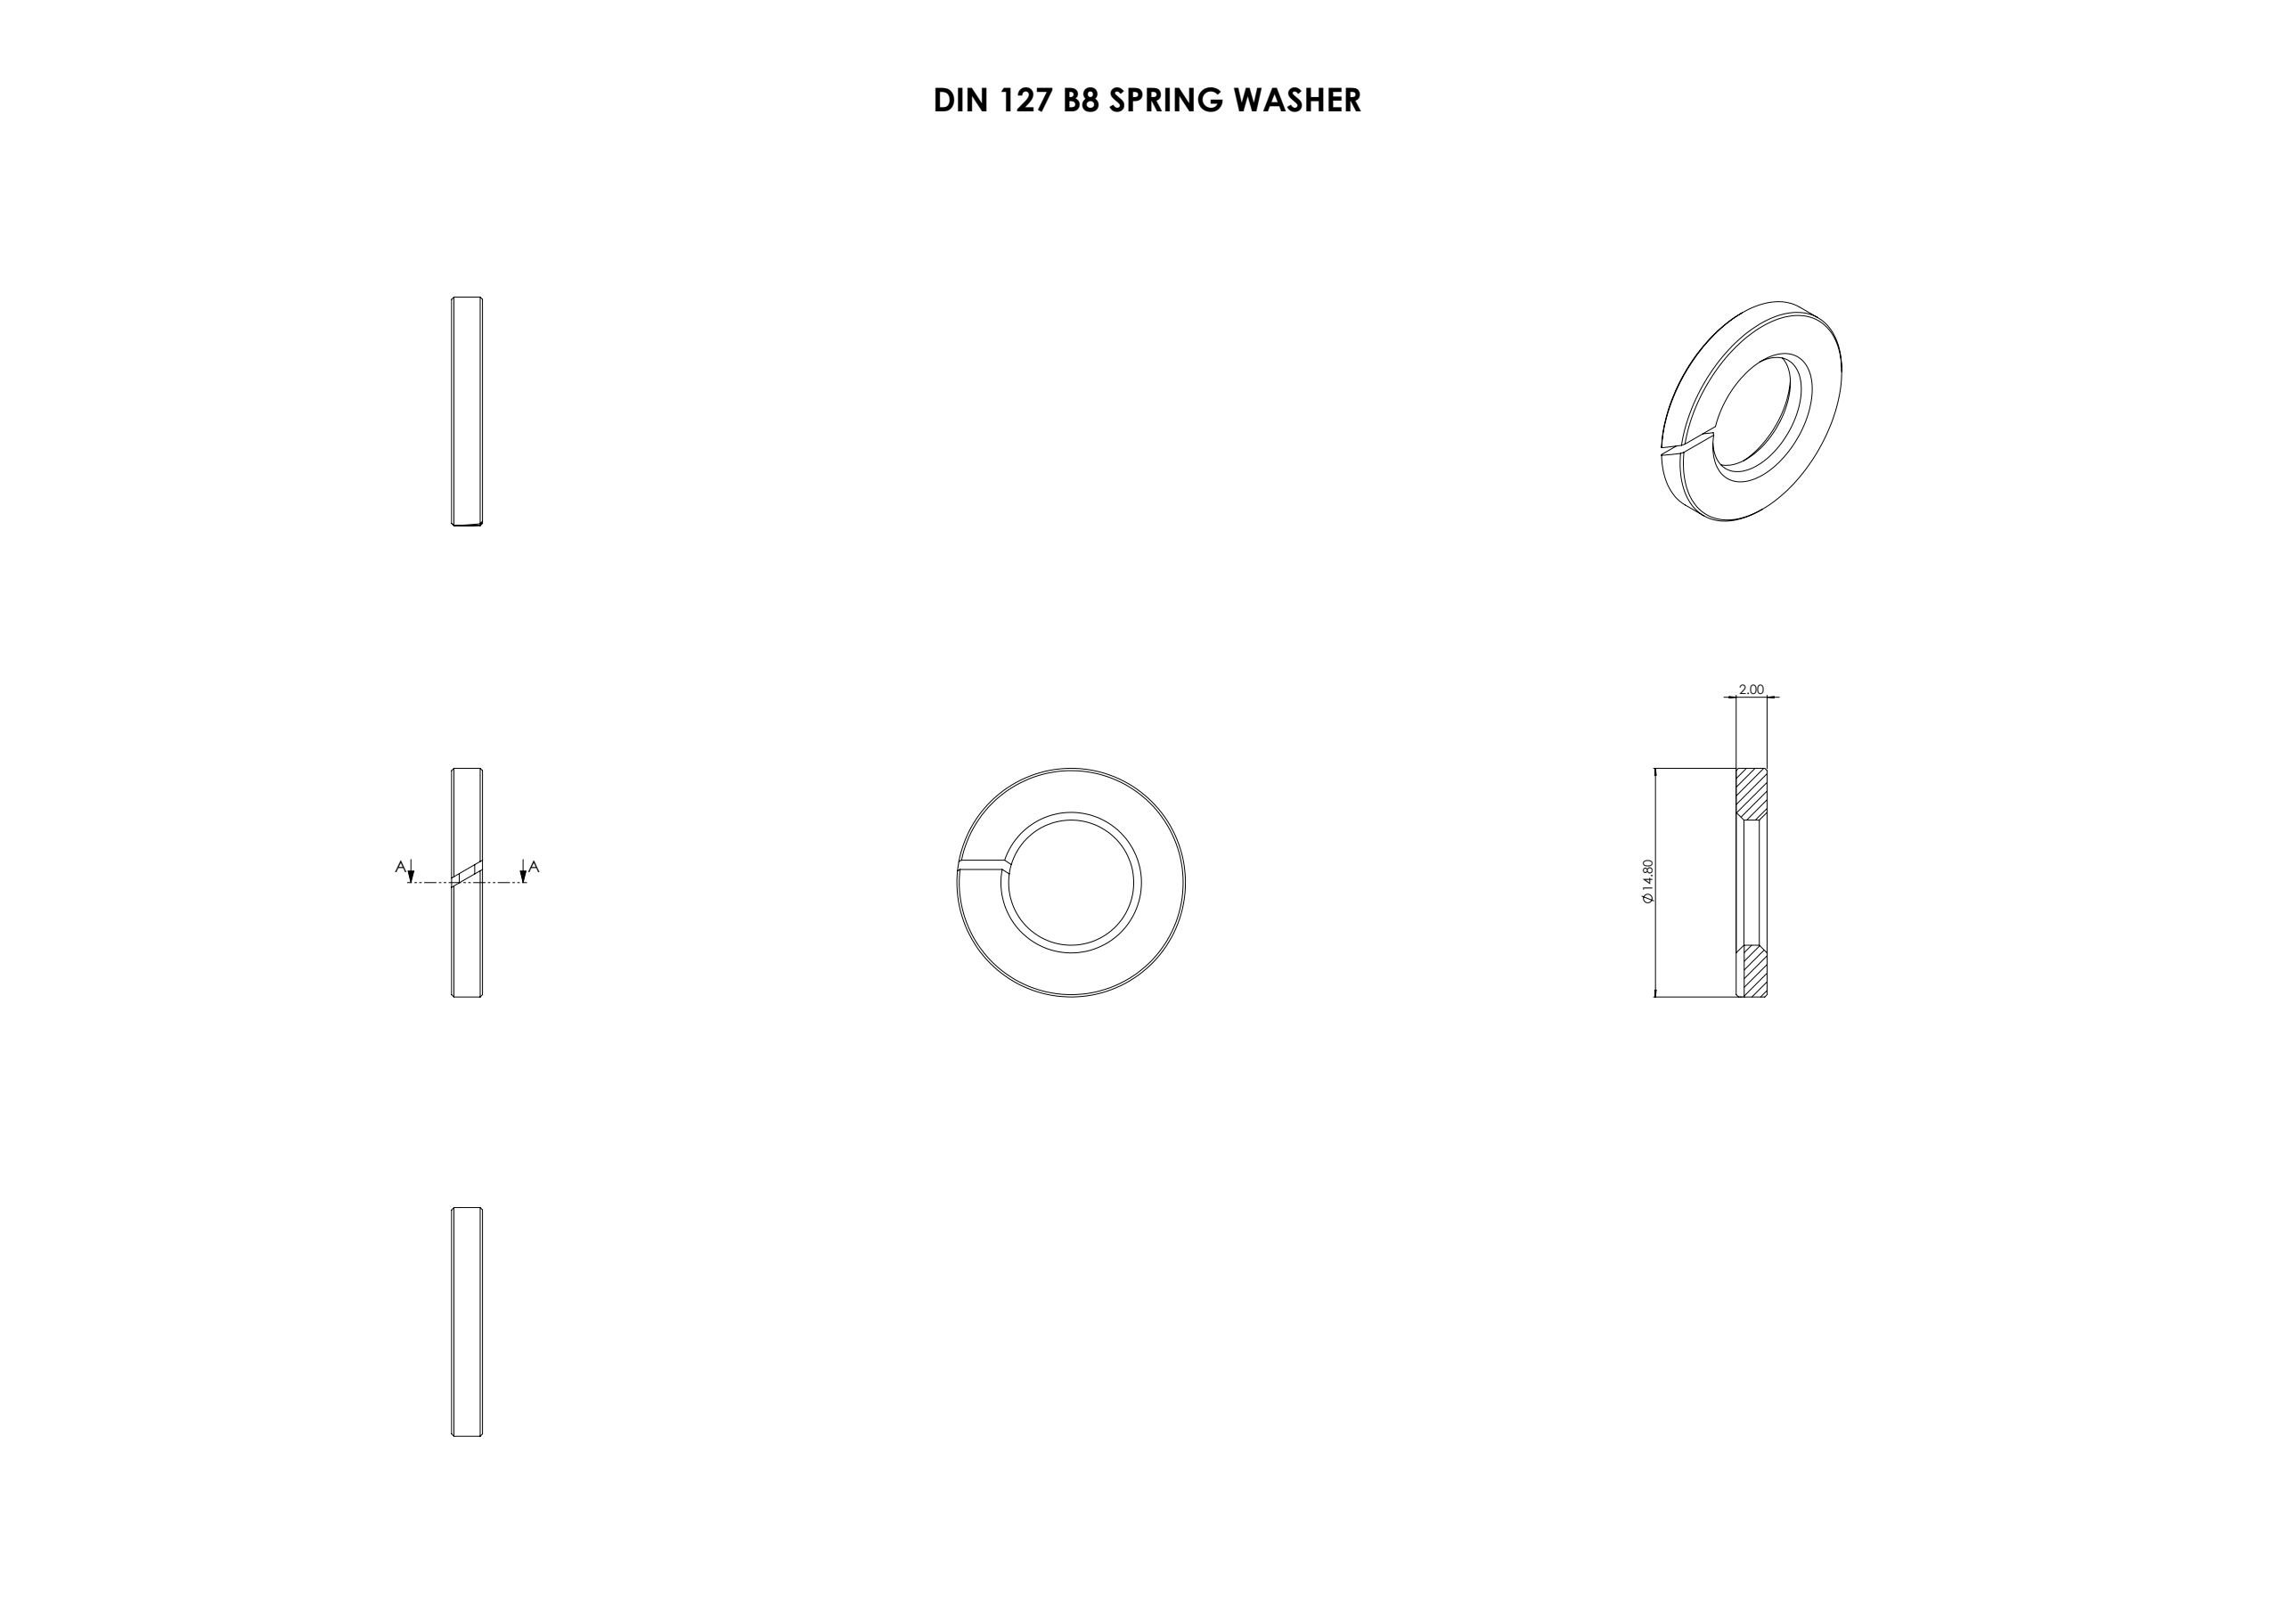
ISO-10303-21;
HEADER;
/* Generated by software containing ST-Developer
 * from STEP Tools, Inc. (www.steptools.com) 
 */

FILE_DESCRIPTION(
/* description */ (''),
/* implementation_level */ '2;1');

FILE_NAME(
/* name */ '13_DIN_127_B8_Spring_Washer.step',
/* time_stamp */ '2026-10-11T08:27:52-07:00',
/* author */ (''),
/* organization */ (''),
/* preprocessor_version */ 'ST-DEVELOPER v20.2',
/* originating_system */ 'Autodesk Translation Framework v15.15.0.0',
/* authorisation */ '');

FILE_SCHEMA (('AUTOMOTIVE_DESIGN { 1 0 10303 214 3 1 1 }'));
ENDSEC;

DATA;
#10=MECHANICAL_DESIGN_GEOMETRIC_PRESENTATION_REPRESENTATION('',(#931),#94301);
#903=SHAPE_REPRESENTATION_RELATIONSHIP('SRR','None',#94383,#917);
#917=ADVANCED_BREP_SHAPE_REPRESENTATION('',(#945),#94299);
#931=STYLED_ITEM('',(#94588),#945);
#945=MANIFOLD_SOLID_BREP('Body1',#51030);
#1284=CYLINDRICAL_SURFACE('',#55289,7.4);
#1285=CYLINDRICAL_SURFACE('',#55301,7.4);
#1286=CYLINDRICAL_SURFACE('',#55309,4.05);
#2156=ELLIPSE('',#55291,14.8,7.4);
#2157=ELLIPSE('',#55294,14.8,7.4);
#2158=ELLIPSE('',#55295,8.1,4.05);
#2159=ELLIPSE('',#55297,8.1,4.05);
#6672=LINE('',#94082,#11200);
#6673=LINE('',#94095,#11201);
#6674=LINE('',#94107,#11202);
#6675=LINE('',#94126,#11203);
#6676=LINE('',#94134,#11204);
#11200=VECTOR('',#68086,7.4);
#11201=VECTOR('',#68095,10.);
#11202=VECTOR('',#68098,10.);
#11203=VECTOR('',#68105,10.);
#11204=VECTOR('',#68106,10.);
#13237=PLANE('',#55293);
#13238=PLANE('',#55296);
#13239=PLANE('',#55305);
#13240=PLANE('',#55313);
#15907=FACE_OUTER_BOUND('',#18672,.T.);
#15908=FACE_OUTER_BOUND('',#18673,.T.);
#15909=FACE_OUTER_BOUND('',#18674,.T.);
#15910=FACE_OUTER_BOUND('',#18675,.T.);
#15911=FACE_OUTER_BOUND('',#18676,.T.);
#15912=FACE_OUTER_BOUND('',#18677,.T.);
#15913=FACE_OUTER_BOUND('',#18678,.T.);
#15914=FACE_OUTER_BOUND('',#18679,.T.);
#15915=FACE_OUTER_BOUND('',#18680,.T.);
#15916=FACE_OUTER_BOUND('',#18681,.T.);
#15917=FACE_OUTER_BOUND('',#18682,.T.);
#18672=EDGE_LOOP('',(#48003,#48004,#48005,#48006));
#18673=EDGE_LOOP('',(#48007,#48008,#48009,#48010,#48011,#48012,#48013,#48014));
#18674=EDGE_LOOP('',(#48015,#48016,#48017,#48018,#48019,#48020,#48021,#48022));
#18675=EDGE_LOOP('',(#48023,#48024,#48025,#48026,#48027));
#18676=EDGE_LOOP('',(#48028,#48029,#48030,#48031));
#18677=EDGE_LOOP('',(#48032,#48033,#48034,#48035,#48036));
#18678=EDGE_LOOP('',(#48037,#48038,#48039,#48040));
#18679=EDGE_LOOP('',(#48041,#48042,#48043,#48044));
#18680=EDGE_LOOP('',(#48045,#48046,#48047,#48048));
#18681=EDGE_LOOP('',(#48049,#48050,#48051,#48052));
#18682=EDGE_LOOP('',(#48053,#48054,#48055,#48056));
#19554=(
BOUNDED_CURVE()
B_SPLINE_CURVE(2,(#94091,#94092,#94093),.UNSPECIFIED.,.F.,.F.)
B_SPLINE_CURVE_WITH_KNOTS((3,3),(0.,0.0721484594100608),.UNSPECIFIED.)
CURVE()
GEOMETRIC_REPRESENTATION_ITEM()
RATIONAL_B_SPLINE_CURVE((1.,1.00124478006548,1.))
REPRESENTATION_ITEM('')
);
#19555=(
BOUNDED_CURVE()
B_SPLINE_CURVE(2,(#94097,#94098,#94099),.UNSPECIFIED.,.F.,.F.)
B_SPLINE_CURVE_WITH_KNOTS((3,3),(0.,0.0242606382665389),.UNSPECIFIED.)
CURVE()
GEOMETRIC_REPRESENTATION_ITEM()
RATIONAL_B_SPLINE_CURVE((1.,1.00003629689575,1.))
REPRESENTATION_ITEM('')
);
#19556=(
BOUNDED_CURVE()
B_SPLINE_CURVE(2,(#94103,#94104,#94105),.UNSPECIFIED.,.F.,.F.)
B_SPLINE_CURVE_WITH_KNOTS((3,3),(0.,0.022659739228849),.UNSPECIFIED.)
CURVE()
GEOMETRIC_REPRESENTATION_ITEM()
RATIONAL_B_SPLINE_CURVE((1.,1.00003502487514,1.))
REPRESENTATION_ITEM('')
);
#19557=(
BOUNDED_CURVE()
B_SPLINE_CURVE(2,(#94109,#94110,#94111),.UNSPECIFIED.,.F.,.F.)
B_SPLINE_CURVE_WITH_KNOTS((3,3),(0.,0.0785853165973684),.UNSPECIFIED.)
CURVE()
GEOMETRIC_REPRESENTATION_ITEM()
RATIONAL_B_SPLINE_CURVE((1.,1.00114268434673,1.))
REPRESENTATION_ITEM('')
);
#19558=(
BOUNDED_CURVE()
B_SPLINE_CURVE(2,(#94116,#94117,#94118),.UNSPECIFIED.,.F.,.F.)
B_SPLINE_CURVE_WITH_KNOTS((3,3),(0.,0.0737421516508094),.UNSPECIFIED.)
CURVE()
GEOMETRIC_REPRESENTATION_ITEM()
RATIONAL_B_SPLINE_CURVE((1.,1.00116107240881,1.))
REPRESENTATION_ITEM('')
);
#19559=(
BOUNDED_CURVE()
B_SPLINE_CURVE(2,(#94122,#94123,#94124),.UNSPECIFIED.,.F.,.F.)
B_SPLINE_CURVE_WITH_KNOTS((3,3),(0.,0.0757335241689913),.UNSPECIFIED.)
CURVE()
GEOMETRIC_REPRESENTATION_ITEM()
RATIONAL_B_SPLINE_CURVE((1.,1.00113125487949,1.))
REPRESENTATION_ITEM('')
);
#19560=(
BOUNDED_CURVE()
B_SPLINE_CURVE(2,(#94127,#94128,#94129),.UNSPECIFIED.,.F.,.F.)
B_SPLINE_CURVE_WITH_KNOTS((3,3),(0.,0.0231191378819049),.UNSPECIFIED.)
CURVE()
GEOMETRIC_REPRESENTATION_ITEM()
RATIONAL_B_SPLINE_CURVE((1.,1.00003499126588,1.))
REPRESENTATION_ITEM('')
);
#19561=(
BOUNDED_CURVE()
B_SPLINE_CURVE(2,(#94131,#94132,#94133),.UNSPECIFIED.,.F.,.F.)
B_SPLINE_CURVE_WITH_KNOTS((3,3),(0.,0.0236194283361202),.UNSPECIFIED.)
CURVE()
GEOMETRIC_REPRESENTATION_ITEM()
RATIONAL_B_SPLINE_CURVE((1.,1.0000353828725,1.))
REPRESENTATION_ITEM('')
);
#20308=CIRCLE('',#55290,7.4);
#20309=CIRCLE('',#55292,7.4);
#20310=CIRCLE('',#55299,7.4);
#20311=CIRCLE('',#55300,7.25);
#20312=CIRCLE('',#55302,7.4);
#20313=CIRCLE('',#55304,7.25);
#20314=CIRCLE('',#55306,4.55);
#20315=CIRCLE('',#55308,4.05);
#20316=CIRCLE('',#55310,4.05);
#20317=CIRCLE('',#55312,4.55);
#25285=VERTEX_POINT('',#94080);
#25286=VERTEX_POINT('',#94081);
#25287=VERTEX_POINT('',#94083);
#25288=VERTEX_POINT('',#94085);
#25289=VERTEX_POINT('',#94089);
#25290=VERTEX_POINT('',#94090);
#25291=VERTEX_POINT('',#94094);
#25292=VERTEX_POINT('',#94096);
#25293=VERTEX_POINT('',#94100);
#25294=VERTEX_POINT('',#94102);
#25295=VERTEX_POINT('',#94106);
#25296=VERTEX_POINT('',#94108);
#25297=VERTEX_POINT('',#94114);
#25298=VERTEX_POINT('',#94115);
#25299=VERTEX_POINT('',#94119);
#25300=VERTEX_POINT('',#94121);
#25301=VERTEX_POINT('',#94125);
#25302=VERTEX_POINT('',#94130);
#32863=EDGE_CURVE('',#25285,#25286,#6672,.T.);
#32864=EDGE_CURVE('',#25287,#25285,#20308,.T.);
#32865=EDGE_CURVE('',#25287,#25288,#2156,.T.);
#32866=EDGE_CURVE('',#25286,#25288,#20309,.T.);
#32867=EDGE_CURVE('',#25289,#25290,#19554,.T.);
#32868=EDGE_CURVE('',#25291,#25289,#6673,.T.);
#32869=EDGE_CURVE('',#25292,#25291,#19555,.T.);
#32870=EDGE_CURVE('',#25293,#25292,#2157,.T.);
#32871=EDGE_CURVE('',#25294,#25293,#19556,.T.);
#32872=EDGE_CURVE('',#25295,#25294,#6674,.T.);
#32873=EDGE_CURVE('',#25296,#25295,#19557,.T.);
#32874=EDGE_CURVE('',#25290,#25296,#2158,.T.);
#32875=EDGE_CURVE('',#25297,#25298,#19558,.T.);
#32876=EDGE_CURVE('',#25299,#25297,#2159,.T.);
#32877=EDGE_CURVE('',#25300,#25299,#19559,.T.);
#32878=EDGE_CURVE('',#25301,#25300,#6675,.T.);
#32879=EDGE_CURVE('',#25288,#25301,#19560,.T.);
#32880=EDGE_CURVE('',#25302,#25287,#19561,.T.);
#32881=EDGE_CURVE('',#25298,#25302,#6676,.T.);
#32882=EDGE_CURVE('',#25293,#25286,#20310,.T.);
#32883=EDGE_CURVE('',#25301,#25294,#20311,.T.);
#32884=EDGE_CURVE('',#25285,#25292,#20312,.T.);
#32885=EDGE_CURVE('',#25291,#25302,#20313,.T.);
#32886=EDGE_CURVE('',#25298,#25289,#20314,.T.);
#32887=EDGE_CURVE('',#25290,#25297,#20315,.T.);
#32888=EDGE_CURVE('',#25299,#25296,#20316,.T.);
#32889=EDGE_CURVE('',#25295,#25300,#20317,.T.);
#48003=ORIENTED_EDGE('',*,*,#32863,.F.);
#48004=ORIENTED_EDGE('',*,*,#32864,.F.);
#48005=ORIENTED_EDGE('',*,*,#32865,.T.);
#48006=ORIENTED_EDGE('',*,*,#32866,.F.);
#48007=ORIENTED_EDGE('',*,*,#32867,.F.);
#48008=ORIENTED_EDGE('',*,*,#32868,.F.);
#48009=ORIENTED_EDGE('',*,*,#32869,.F.);
#48010=ORIENTED_EDGE('',*,*,#32870,.F.);
#48011=ORIENTED_EDGE('',*,*,#32871,.F.);
#48012=ORIENTED_EDGE('',*,*,#32872,.F.);
#48013=ORIENTED_EDGE('',*,*,#32873,.F.);
#48014=ORIENTED_EDGE('',*,*,#32874,.F.);
#48015=ORIENTED_EDGE('',*,*,#32875,.F.);
#48016=ORIENTED_EDGE('',*,*,#32876,.F.);
#48017=ORIENTED_EDGE('',*,*,#32877,.F.);
#48018=ORIENTED_EDGE('',*,*,#32878,.F.);
#48019=ORIENTED_EDGE('',*,*,#32879,.F.);
#48020=ORIENTED_EDGE('',*,*,#32865,.F.);
#48021=ORIENTED_EDGE('',*,*,#32880,.F.);
#48022=ORIENTED_EDGE('',*,*,#32881,.F.);
#48023=ORIENTED_EDGE('',*,*,#32871,.T.);
#48024=ORIENTED_EDGE('',*,*,#32882,.T.);
#48025=ORIENTED_EDGE('',*,*,#32866,.T.);
#48026=ORIENTED_EDGE('',*,*,#32879,.T.);
#48027=ORIENTED_EDGE('',*,*,#32883,.T.);
#48028=ORIENTED_EDGE('',*,*,#32863,.T.);
#48029=ORIENTED_EDGE('',*,*,#32882,.F.);
#48030=ORIENTED_EDGE('',*,*,#32870,.T.);
#48031=ORIENTED_EDGE('',*,*,#32884,.F.);
#48032=ORIENTED_EDGE('',*,*,#32869,.T.);
#48033=ORIENTED_EDGE('',*,*,#32885,.T.);
#48034=ORIENTED_EDGE('',*,*,#32880,.T.);
#48035=ORIENTED_EDGE('',*,*,#32864,.T.);
#48036=ORIENTED_EDGE('',*,*,#32884,.T.);
#48037=ORIENTED_EDGE('',*,*,#32868,.T.);
#48038=ORIENTED_EDGE('',*,*,#32886,.F.);
#48039=ORIENTED_EDGE('',*,*,#32881,.T.);
#48040=ORIENTED_EDGE('',*,*,#32885,.F.);
#48041=ORIENTED_EDGE('',*,*,#32867,.T.);
#48042=ORIENTED_EDGE('',*,*,#32887,.T.);
#48043=ORIENTED_EDGE('',*,*,#32875,.T.);
#48044=ORIENTED_EDGE('',*,*,#32886,.T.);
#48045=ORIENTED_EDGE('',*,*,#32874,.T.);
#48046=ORIENTED_EDGE('',*,*,#32888,.F.);
#48047=ORIENTED_EDGE('',*,*,#32876,.T.);
#48048=ORIENTED_EDGE('',*,*,#32887,.F.);
#48049=ORIENTED_EDGE('',*,*,#32873,.T.);
#48050=ORIENTED_EDGE('',*,*,#32889,.T.);
#48051=ORIENTED_EDGE('',*,*,#32877,.T.);
#48052=ORIENTED_EDGE('',*,*,#32888,.T.);
#48053=ORIENTED_EDGE('',*,*,#32872,.T.);
#48054=ORIENTED_EDGE('',*,*,#32883,.F.);
#48055=ORIENTED_EDGE('',*,*,#32878,.T.);
#48056=ORIENTED_EDGE('',*,*,#32889,.F.);
#48328=CONICAL_SURFACE('',#55298,7.325,0.785398163397449);
#48329=CONICAL_SURFACE('',#55303,7.325,0.785398163397448);
#48330=CONICAL_SURFACE('',#55307,4.3,0.785398163397448);
#48331=CONICAL_SURFACE('',#55311,4.3,0.785398163397448);
#50994=ADVANCED_FACE('',(#15907),#1284,.T.);
#50995=ADVANCED_FACE('',(#15908),#13237,.F.);
#50996=ADVANCED_FACE('',(#15909),#13238,.F.);
#50997=ADVANCED_FACE('',(#15910),#48328,.T.);
#50998=ADVANCED_FACE('',(#15911),#1285,.T.);
#50999=ADVANCED_FACE('',(#15912),#48329,.T.);
#51000=ADVANCED_FACE('',(#15913),#13239,.T.);
#51001=ADVANCED_FACE('',(#15914),#48330,.F.);
#51002=ADVANCED_FACE('',(#15915),#1286,.F.);
#51003=ADVANCED_FACE('',(#15916),#48331,.F.);
#51004=ADVANCED_FACE('',(#15917),#13240,.T.);
#51030=CLOSED_SHELL('',(#50994,#50995,#50996,#50997,#50998,#50999,#51000,
#51001,#51002,#51003,#51004));
#55288=AXIS2_PLACEMENT_3D('',#94078,#68082,#68083);
#55289=AXIS2_PLACEMENT_3D('',#94079,#68084,#68085);
#55290=AXIS2_PLACEMENT_3D('',#94084,#68087,#68088);
#55291=AXIS2_PLACEMENT_3D('',#94086,#68089,#68090);
#55292=AXIS2_PLACEMENT_3D('',#94087,#68091,#68092);
#55293=AXIS2_PLACEMENT_3D('',#94088,#68093,#68094);
#55294=AXIS2_PLACEMENT_3D('',#94101,#68096,#68097);
#55295=AXIS2_PLACEMENT_3D('',#94112,#68099,#68100);
#55296=AXIS2_PLACEMENT_3D('',#94113,#68101,#68102);
#55297=AXIS2_PLACEMENT_3D('',#94120,#68103,#68104);
#55298=AXIS2_PLACEMENT_3D('',#94135,#68107,#68108);
#55299=AXIS2_PLACEMENT_3D('',#94136,#68109,#68110);
#55300=AXIS2_PLACEMENT_3D('',#94137,#68111,#68112);
#55301=AXIS2_PLACEMENT_3D('',#94138,#68113,#68114);
#55302=AXIS2_PLACEMENT_3D('',#94139,#68115,#68116);
#55303=AXIS2_PLACEMENT_3D('',#94140,#68117,#68118);
#55304=AXIS2_PLACEMENT_3D('',#94141,#68119,#68120);
#55305=AXIS2_PLACEMENT_3D('',#94142,#68121,#68122);
#55306=AXIS2_PLACEMENT_3D('',#94143,#68123,#68124);
#55307=AXIS2_PLACEMENT_3D('',#94144,#68125,#68126);
#55308=AXIS2_PLACEMENT_3D('',#94145,#68127,#68128);
#55309=AXIS2_PLACEMENT_3D('',#94146,#68129,#68130);
#55310=AXIS2_PLACEMENT_3D('',#94147,#68131,#68132);
#55311=AXIS2_PLACEMENT_3D('',#94148,#68133,#68134);
#55312=AXIS2_PLACEMENT_3D('',#94149,#68135,#68136);
#55313=AXIS2_PLACEMENT_3D('',#94150,#68137,#68138);
#68082=DIRECTION('axis',(0.,0.,1.));
#68083=DIRECTION('refdir',(1.,0.,0.));
#68084=DIRECTION('center_axis',(1.,0.,0.));
#68085=DIRECTION('ref_axis',(0.,1.,0.));
#68086=DIRECTION('',(-1.,0.,0.));
#68087=DIRECTION('center_axis',(1.,0.,0.));
#68088=DIRECTION('ref_axis',(0.,-1.,0.));
#68089=DIRECTION('center_axis',(0.5,-0.866025403784439,0.));
#68090=DIRECTION('ref_axis',(0.866025403784439,0.5,0.));
#68091=DIRECTION('center_axis',(-1.,0.,0.));
#68092=DIRECTION('ref_axis',(0.,-1.,0.));
#68093=DIRECTION('center_axis',(-0.5,0.866025403784439,0.));
#68094=DIRECTION('ref_axis',(-0.866025403784439,-0.5,0.));
#68095=DIRECTION('',(0.,0.,-1.));
#68096=DIRECTION('center_axis',(-0.5,0.866025403784439,0.));
#68097=DIRECTION('ref_axis',(0.866025403784439,0.5,0.));
#68098=DIRECTION('',(0.,0.,1.));
#68099=DIRECTION('center_axis',(0.5,-0.866025403784439,0.));
#68100=DIRECTION('ref_axis',(0.866025403784439,0.5,0.));
#68101=DIRECTION('center_axis',(0.5,-0.866025403784439,0.));
#68102=DIRECTION('ref_axis',(0.866025403784439,0.5,0.));
#68103=DIRECTION('center_axis',(-0.5,0.866025403784439,0.));
#68104=DIRECTION('ref_axis',(0.866025403784439,0.5,0.));
#68105=DIRECTION('',(0.,0.,-1.));
#68106=DIRECTION('',(0.,0.,1.));
#68107=DIRECTION('center_axis',(1.,0.,0.));
#68108=DIRECTION('ref_axis',(0.,-0.00627477638988747,-0.999980313396847));
#68109=DIRECTION('center_axis',(-1.,0.,0.));
#68110=DIRECTION('ref_axis',(0.,-1.,0.));
#68111=DIRECTION('center_axis',(1.,0.,0.));
#68112=DIRECTION('ref_axis',(0.,-1.,0.));
#68113=DIRECTION('center_axis',(1.,0.,0.));
#68114=DIRECTION('ref_axis',(0.,1.,0.));
#68115=DIRECTION('center_axis',(1.,0.,0.));
#68116=DIRECTION('ref_axis',(0.,-1.,0.));
#68117=DIRECTION('center_axis',(-1.,0.,0.));
#68118=DIRECTION('ref_axis',(0.,-0.151470903394779,-0.988461716721882));
#68119=DIRECTION('center_axis',(-1.,0.,0.));
#68120=DIRECTION('ref_axis',(0.,-1.,0.));
#68121=DIRECTION('center_axis',(1.,0.,0.));
#68122=DIRECTION('ref_axis',(0.,0.,-1.));
#68123=DIRECTION('center_axis',(1.,0.,0.));
#68124=DIRECTION('ref_axis',(0.,-1.,0.));
#68125=DIRECTION('center_axis',(1.,0.,0.));
#68126=DIRECTION('ref_axis',(0.,-0.238193136410173,-0.971217807583389));
#68127=DIRECTION('center_axis',(-1.,0.,0.));
#68128=DIRECTION('ref_axis',(0.,-1.,0.));
#68129=DIRECTION('center_axis',(1.,0.,0.));
#68130=DIRECTION('ref_axis',(0.,-0.142556190914054,-0.989786710575605));
#68131=DIRECTION('center_axis',(1.,0.,0.));
#68132=DIRECTION('ref_axis',(0.,-1.,0.));
#68133=DIRECTION('center_axis',(-1.,0.,0.));
#68134=DIRECTION('ref_axis',(0.,-0.0315875774899171,-0.999500987967655));
#68135=DIRECTION('center_axis',(-1.,0.,0.));
#68136=DIRECTION('ref_axis',(0.,-1.,0.));
#68137=DIRECTION('center_axis',(-1.,0.,0.));
#68138=DIRECTION('ref_axis',(0.,0.,1.));
#94078=CARTESIAN_POINT('',(0.,0.,0.));
#94079=CARTESIAN_POINT('Origin',(1.,0.,0.));
#94080=CARTESIAN_POINT('',(1.85,-7.4,-9.06238631369041E-16));
#94081=CARTESIAN_POINT('',(0.15,-7.4,-9.06238631369041E-16));
#94082=CARTESIAN_POINT('',(1.,-7.4,-9.06238631369041E-16));
#94083=CARTESIAN_POINT('',(1.85,0.768097998000808,7.36002890384726));
#94084=CARTESIAN_POINT('Origin',(1.85,0.,0.));
#94085=CARTESIAN_POINT('',(0.15,-0.213397459621556,7.39692243600182));
#94086=CARTESIAN_POINT('Origin',(0.519615242270663,0.,0.));
#94087=CARTESIAN_POINT('Origin',(0.15,0.,0.));
#94088=CARTESIAN_POINT('Origin',(2.2,1.57017059221718,0.));
#94089=CARTESIAN_POINT('',(2.,1.45470053837925,4.31118850708701));
#94090=CARTESIAN_POINT('',(1.5,1.16602540378444,3.87851579315198));
#94091=CARTESIAN_POINT('Ctrl Pts',(2.,1.45470053837925,4.31118850708701));
#94092=CARTESIAN_POINT('Ctrl Pts',(1.73679217533305,1.30273742995497,4.08467677256398));
#94093=CARTESIAN_POINT('Ctrl Pts',(1.5,1.16602540378444,3.87851579315198));
#94094=CARTESIAN_POINT('',(2.,1.45470053837925,7.10255914045347));
#94095=CARTESIAN_POINT('',(2.,1.45470053837925,0.));
#94096=CARTESIAN_POINT('',(1.85,1.36809799800081,7.2724347963984));
#94097=CARTESIAN_POINT('Ctrl Pts',(1.85,1.36809799800081,7.2724347963984));
#94098=CARTESIAN_POINT('Ctrl Pts',(1.92588630814391,1.4119109784355,7.18697522907551));
#94099=CARTESIAN_POINT('Ctrl Pts',(2.,1.45470053837925,7.10255914045347));
#94100=CARTESIAN_POINT('',(0.15,0.386602540378444,7.3898943480792));
#94101=CARTESIAN_POINT('Origin',(-0.519615242270663,0.,0.));
#94102=CARTESIAN_POINT('',(0.,0.3,7.24379044423567));
#94103=CARTESIAN_POINT('Ctrl Pts',(2.86229373536173E-16,0.3,7.24379044423567));
#94104=CARTESIAN_POINT('Ctrl Pts',(0.0742511938739692,0.342868946770787,
7.31632987999105));
#94105=CARTESIAN_POINT('Ctrl Pts',(0.15,0.386602540378444,7.3898943480792));
#94106=CARTESIAN_POINT('',(0.,0.3,4.54009911786075));
#94107=CARTESIAN_POINT('',(5.55111512312578E-16,0.300000000000001,0.));
#94108=CARTESIAN_POINT('',(0.5,0.588675134594813,4.0069890923123));
#94109=CARTESIAN_POINT('Ctrl Pts',(0.5,0.588675134594813,4.0069890923123));
#94110=CARTESIAN_POINT('Ctrl Pts',(0.26559332290833,0.453340376476092,4.26379419596142));
#94111=CARTESIAN_POINT('Ctrl Pts',(3.12250225675825E-16,0.3,4.54009911786075));
#94112=CARTESIAN_POINT('Origin',(-0.519615242270663,0.,0.));
#94113=CARTESIAN_POINT('Origin',(-0.2,-0.415470053837925,0.));
#94114=CARTESIAN_POINT('',(1.5,0.566025403784439,4.01025126921876));
#94115=CARTESIAN_POINT('',(2.,0.854700538379251,4.4690029077742));
#94116=CARTESIAN_POINT('Ctrl Pts',(1.5,0.566025403784439,4.01025126921876));
#94117=CARTESIAN_POINT('Ctrl Pts',(1.73647429275706,0.702553900364154,4.22979918009891));
#94118=CARTESIAN_POINT('Ctrl Pts',(2.,0.854700538379252,4.4690029077742));
#94119=CARTESIAN_POINT('',(0.5,-0.011324865405187,4.04998416631764));
#94120=CARTESIAN_POINT('Origin',(0.519615242270663,0.,0.));
#94121=CARTESIAN_POINT('',(0.,-0.3,4.54009911786075));
#94122=CARTESIAN_POINT('Ctrl Pts',(0.,-0.3,4.54009911786075));
#94123=CARTESIAN_POINT('Ctrl Pts',(0.264263975543855,-0.147427122582635,
4.28534053319701));
#94124=CARTESIAN_POINT('Ctrl Pts',(0.5,-0.011324865405187,4.04998416631764));
#94125=CARTESIAN_POINT('',(0.,-0.3,7.24379044423567));
#94126=CARTESIAN_POINT('',(2.77555756156289E-16,-0.3,0.));
#94127=CARTESIAN_POINT('Ctrl Pts',(0.15,-0.213397459621556,7.39692243600182));
#94128=CARTESIAN_POINT('Ctrl Pts',(0.0742155505352446,-0.25715163192042,
7.31984416998126));
#94129=CARTESIAN_POINT('Ctrl Pts',(8.67361737988404E-18,-0.3,7.24379044423567));
#94130=CARTESIAN_POINT('',(2.,0.854700538379251,7.19944351944608));
#94131=CARTESIAN_POINT('Ctrl Pts',(2.,0.854700538379252,7.19944351944608));
#94132=CARTESIAN_POINT('Ctrl Pts',(1.92582722117148,0.811876864556063,7.27922108309076));
#94133=CARTESIAN_POINT('Ctrl Pts',(1.85,0.768097998000808,7.36002890384726));
#94134=CARTESIAN_POINT('',(2.,0.854700538379251,0.));
#94135=CARTESIAN_POINT('Origin',(0.075,0.,0.));
#94136=CARTESIAN_POINT('Origin',(0.15,0.,0.));
#94137=CARTESIAN_POINT('Origin',(0.,0.,0.));
#94138=CARTESIAN_POINT('Origin',(1.,0.,0.));
#94139=CARTESIAN_POINT('Origin',(1.85,0.,0.));
#94140=CARTESIAN_POINT('Origin',(1.925,0.,0.));
#94141=CARTESIAN_POINT('Origin',(2.,0.,0.));
#94142=CARTESIAN_POINT('Origin',(2.,4.05,0.));
#94143=CARTESIAN_POINT('Origin',(2.,0.,0.));
#94144=CARTESIAN_POINT('Origin',(1.75,0.,0.));
#94145=CARTESIAN_POINT('Origin',(1.5,0.,0.));
#94146=CARTESIAN_POINT('Origin',(1.,0.,0.));
#94147=CARTESIAN_POINT('Origin',(0.5,0.,0.));
#94148=CARTESIAN_POINT('Origin',(0.25,0.,0.));
#94149=CARTESIAN_POINT('Origin',(0.,0.,0.));
#94150=CARTESIAN_POINT('Origin',(0.,7.4,0.));
#94283=UNCERTAINTY_MEASURE_WITH_UNIT(LENGTH_MEASURE(0.01),#94302,
'DISTANCE_ACCURACY_VALUE',
'Maximum model space distance between geometric entities at asserted c
onnectivities');
#94285=UNCERTAINTY_MEASURE_WITH_UNIT(LENGTH_MEASURE(0.01),#94302,
'DISTANCE_ACCURACY_VALUE',
'Maximum model space distance between geometric entities at asserted c
onnectivities');
#94299=(
GEOMETRIC_REPRESENTATION_CONTEXT(3)
GLOBAL_UNCERTAINTY_ASSIGNED_CONTEXT((#94283))
GLOBAL_UNIT_ASSIGNED_CONTEXT((#94302,#94304,#94305))
REPRESENTATION_CONTEXT('','3D')
);
#94301=(
GEOMETRIC_REPRESENTATION_CONTEXT(3)
GLOBAL_UNCERTAINTY_ASSIGNED_CONTEXT((#94285))
GLOBAL_UNIT_ASSIGNED_CONTEXT((#94302,#94304,#94305))
REPRESENTATION_CONTEXT('','3D')
);
#94302=(
LENGTH_UNIT()
NAMED_UNIT(*)
SI_UNIT(.MILLI.,.METRE.)
);
#94304=(
NAMED_UNIT(*)
PLANE_ANGLE_UNIT()
SI_UNIT($,.RADIAN.)
);
#94305=(
NAMED_UNIT(*)
SI_UNIT($,.STERADIAN.)
SOLID_ANGLE_UNIT()
);
#94319=SHAPE_DEFINITION_REPRESENTATION(#94334,#94383);
#94334=PRODUCT_DEFINITION_SHAPE('',$,#94399);
#94383=SHAPE_REPRESENTATION('',(#55288),#94299);
#94385=PRODUCT_DEFINITION_CONTEXT('part definition',#94432,'design');
#94399=PRODUCT_DEFINITION('2026-10-11-08-26-49-607',
'13_DIN_127_B8_Spring_Washer',#94414,#94385);
#94414=PRODUCT_DEFINITION_FORMATION('',$,#94447);
#94432=APPLICATION_CONTEXT(
'Core Data for Automotive Mechanical Design Process');
#94433=PRODUCT_CONTEXT('part definition',#94432,'mechanical');
#94447=PRODUCT('2026-10-11-08-26-49-607','13_DIN_127_B8_Spring_Washer',
$,(#94433));
#94582=COLOUR_RGB('Black',0.12,0.14,0.17);
#94583=FILL_AREA_STYLE_COLOUR('',#94582);
#94584=FILL_AREA_STYLE('',(#94583));
#94585=SURFACE_STYLE_FILL_AREA(#94584);
#94586=SURFACE_SIDE_STYLE('',(#94585));
#94587=SURFACE_STYLE_USAGE(.BOTH.,#94586);
#94588=PRESENTATION_STYLE_ASSIGNMENT((#94587));
ENDSEC;
END-ISO-10303-21;
